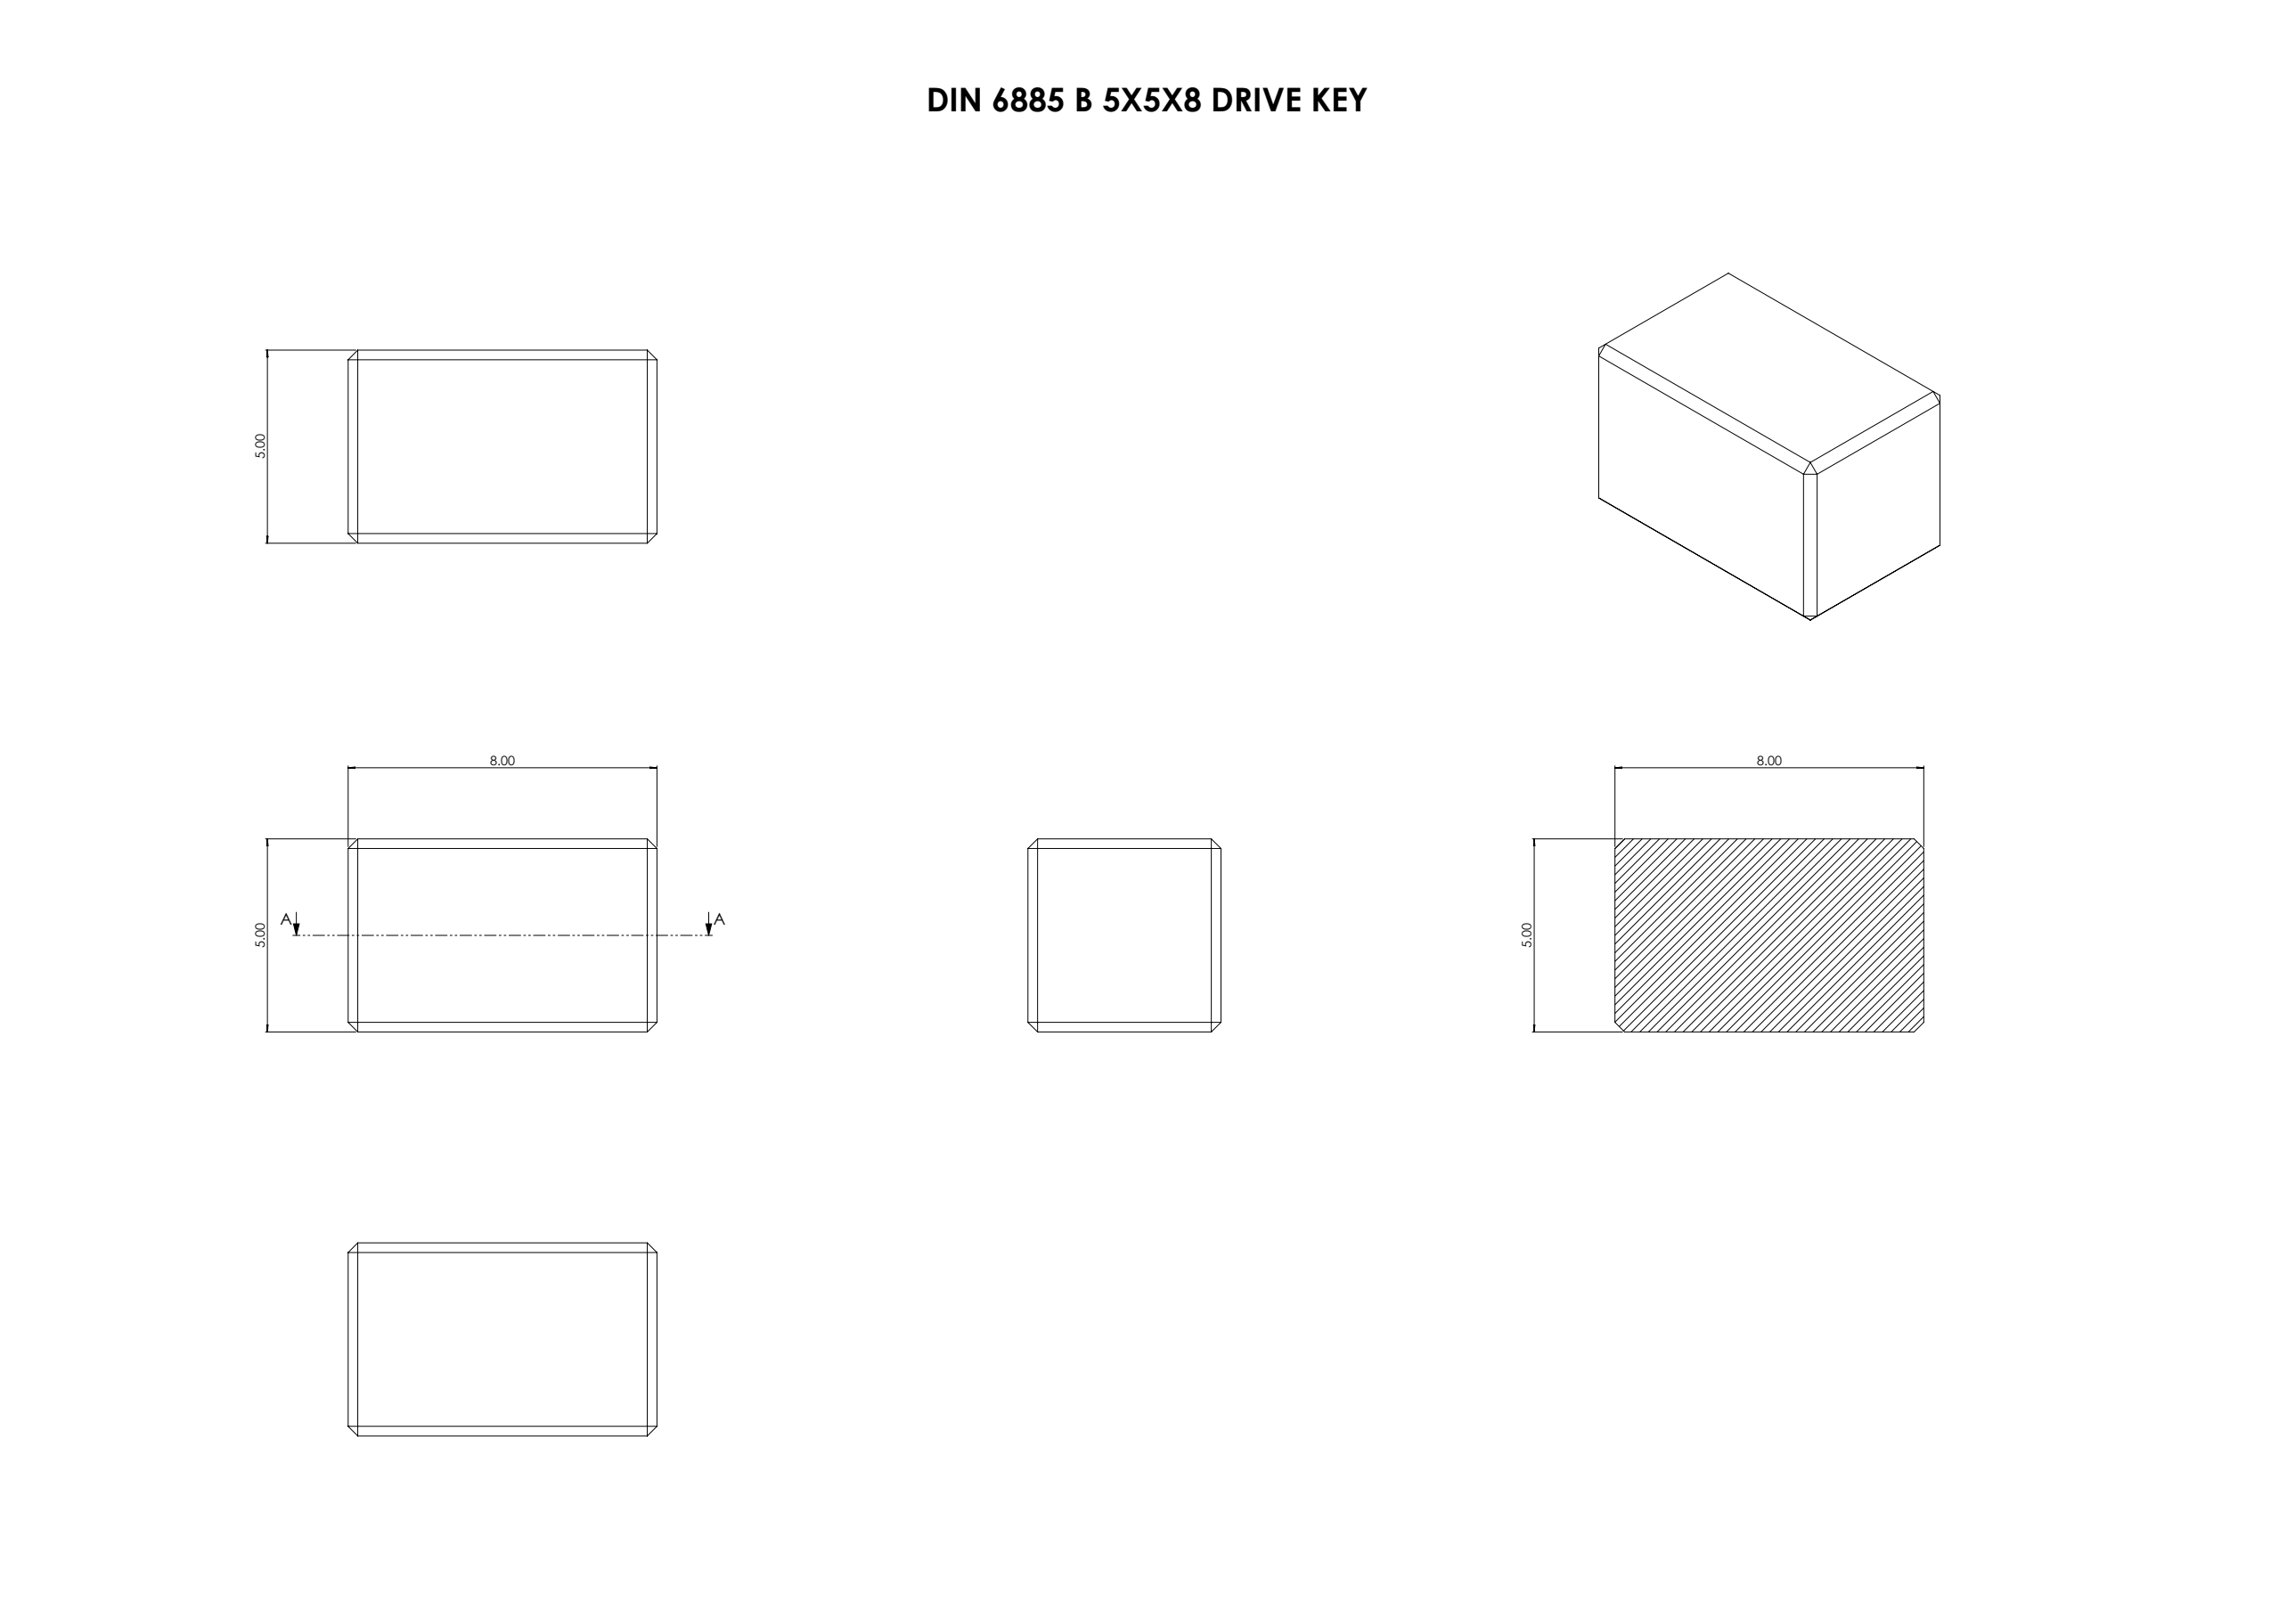
ISO-10303-21;
HEADER;
/* Generated by software containing ST-Developer
 * from STEP Tools, Inc. (www.steptools.com) 
 */

FILE_DESCRIPTION(
/* description */ (''),
/* implementation_level */ '2;1');

FILE_NAME(
/* name */ '10_DIN_6885_B_5x5x8_Drive_Key.step',
/* time_stamp */ '2026-10-24T13:41:11-07:00',
/* author */ (''),
/* organization */ (''),
/* preprocessor_version */ 'ST-DEVELOPER v20.2',
/* originating_system */ 'Autodesk Translation Framework v15.15.0.0',
/* authorisation */ '');

FILE_SCHEMA (('AUTOMOTIVE_DESIGN { 1 0 10303 214 3 1 1 }'));
ENDSEC;

DATA;
#10=MECHANICAL_DESIGN_GEOMETRIC_PRESENTATION_REPRESENTATION('',(#130),#12813);
#110=SHAPE_REPRESENTATION_RELATIONSHIP('SRR','None',#12863,#120);
#120=ADVANCED_BREP_SHAPE_REPRESENTATION('',(#140),#12812);
#130=STYLED_ITEM('',(#12974),#140);
#140=MANIFOLD_SOLID_BREP('Body1',#4393);
#232=PLANE('',#4965);
#233=PLANE('',#4966);
#234=PLANE('',#4967);
#235=PLANE('',#4968);
#236=PLANE('',#4969);
#237=PLANE('',#4970);
#238=PLANE('',#4971);
#239=PLANE('',#4972);
#240=PLANE('',#4973);
#241=PLANE('',#4974);
#242=PLANE('',#4975);
#243=PLANE('',#4976);
#244=PLANE('',#4977);
#245=PLANE('',#4978);
#246=PLANE('',#4979);
#247=PLANE('',#4980);
#248=PLANE('',#4981);
#249=PLANE('',#4982);
#250=PLANE('',#4983);
#251=PLANE('',#4984);
#252=PLANE('',#4985);
#253=PLANE('',#4986);
#254=PLANE('',#4987);
#255=PLANE('',#4988);
#256=PLANE('',#4989);
#257=PLANE('',#4990);
#568=FACE_OUTER_BOUND('',#866,.T.);
#569=FACE_OUTER_BOUND('',#867,.T.);
#570=FACE_OUTER_BOUND('',#868,.T.);
#571=FACE_OUTER_BOUND('',#869,.T.);
#572=FACE_OUTER_BOUND('',#870,.T.);
#573=FACE_OUTER_BOUND('',#871,.T.);
#574=FACE_OUTER_BOUND('',#872,.T.);
#575=FACE_OUTER_BOUND('',#873,.T.);
#576=FACE_OUTER_BOUND('',#874,.T.);
#577=FACE_OUTER_BOUND('',#875,.T.);
#578=FACE_OUTER_BOUND('',#876,.T.);
#579=FACE_OUTER_BOUND('',#877,.T.);
#580=FACE_OUTER_BOUND('',#878,.T.);
#581=FACE_OUTER_BOUND('',#879,.T.);
#582=FACE_OUTER_BOUND('',#880,.T.);
#583=FACE_OUTER_BOUND('',#881,.T.);
#584=FACE_OUTER_BOUND('',#882,.T.);
#585=FACE_OUTER_BOUND('',#883,.T.);
#586=FACE_OUTER_BOUND('',#884,.T.);
#587=FACE_OUTER_BOUND('',#885,.T.);
#588=FACE_OUTER_BOUND('',#886,.T.);
#589=FACE_OUTER_BOUND('',#887,.T.);
#590=FACE_OUTER_BOUND('',#888,.T.);
#591=FACE_OUTER_BOUND('',#889,.T.);
#592=FACE_OUTER_BOUND('',#890,.T.);
#593=FACE_OUTER_BOUND('',#891,.T.);
#866=EDGE_LOOP('',(#3933,#3934,#3935));
#867=EDGE_LOOP('',(#3936,#3937,#3938));
#868=EDGE_LOOP('',(#3939,#3940,#3941));
#869=EDGE_LOOP('',(#3942,#3943,#3944));
#870=EDGE_LOOP('',(#3945,#3946,#3947,#3948));
#871=EDGE_LOOP('',(#3949,#3950,#3951));
#872=EDGE_LOOP('',(#3952,#3953,#3954));
#873=EDGE_LOOP('',(#3955,#3956,#3957,#3958));
#874=EDGE_LOOP('',(#3959,#3960,#3961));
#875=EDGE_LOOP('',(#3962,#3963,#3964,#3965));
#876=EDGE_LOOP('',(#3966,#3967,#3968,#3969));
#877=EDGE_LOOP('',(#3970,#3971,#3972));
#878=EDGE_LOOP('',(#3973,#3974,#3975,#3976));
#879=EDGE_LOOP('',(#3977,#3978,#3979,#3980));
#880=EDGE_LOOP('',(#3981,#3982,#3983,#3984));
#881=EDGE_LOOP('',(#3985,#3986,#3987,#3988));
#882=EDGE_LOOP('',(#3989,#3990,#3991,#3992));
#883=EDGE_LOOP('',(#3993,#3994,#3995,#3996));
#884=EDGE_LOOP('',(#3997,#3998,#3999,#4000));
#885=EDGE_LOOP('',(#4001,#4002,#4003,#4004));
#886=EDGE_LOOP('',(#4005,#4006,#4007,#4008));
#887=EDGE_LOOP('',(#4009,#4010,#4011,#4012));
#888=EDGE_LOOP('',(#4013,#4014,#4015,#4016));
#889=EDGE_LOOP('',(#4017,#4018,#4019,#4020));
#890=EDGE_LOOP('',(#4021,#4022,#4023,#4024));
#891=EDGE_LOOP('',(#4025,#4026,#4027,#4028));
#1305=LINE('',#12682,#1535);
#1306=LINE('',#12684,#1536);
#1307=LINE('',#12685,#1537);
#1308=LINE('',#12689,#1538);
#1309=LINE('',#12691,#1539);
#1310=LINE('',#12692,#1540);
#1311=LINE('',#12696,#1541);
#1312=LINE('',#12698,#1542);
#1313=LINE('',#12699,#1543);
#1314=LINE('',#12703,#1544);
#1315=LINE('',#12705,#1545);
#1316=LINE('',#12706,#1546);
#1317=LINE('',#12708,#1547);
#1318=LINE('',#12709,#1548);
#1319=LINE('',#12713,#1549);
#1320=LINE('',#12715,#1550);
#1321=LINE('',#12716,#1551);
#1322=LINE('',#12720,#1552);
#1323=LINE('',#12722,#1553);
#1324=LINE('',#12723,#1554);
#1325=LINE('',#12725,#1555);
#1326=LINE('',#12726,#1556);
#1327=LINE('',#12730,#1557);
#1328=LINE('',#12732,#1558);
#1329=LINE('',#12733,#1559);
#1330=LINE('',#12735,#1560);
#1331=LINE('',#12736,#1561);
#1332=LINE('',#12738,#1562);
#1333=LINE('',#12739,#1563);
#1334=LINE('',#12743,#1564);
#1335=LINE('',#12745,#1565);
#1336=LINE('',#12746,#1566);
#1337=LINE('',#12748,#1567);
#1338=LINE('',#12749,#1568);
#1339=LINE('',#12751,#1569);
#1340=LINE('',#12752,#1570);
#1341=LINE('',#12754,#1571);
#1342=LINE('',#12755,#1572);
#1343=LINE('',#12757,#1573);
#1344=LINE('',#12758,#1574);
#1345=LINE('',#12760,#1575);
#1346=LINE('',#12761,#1576);
#1347=LINE('',#12763,#1577);
#1348=LINE('',#12764,#1578);
#1349=LINE('',#12766,#1579);
#1350=LINE('',#12767,#1580);
#1351=LINE('',#12769,#1581);
#1352=LINE('',#12770,#1582);
#1535=VECTOR('',#6108,10.);
#1536=VECTOR('',#6109,10.);
#1537=VECTOR('',#6110,10.);
#1538=VECTOR('',#6113,10.);
#1539=VECTOR('',#6114,10.);
#1540=VECTOR('',#6115,10.);
#1541=VECTOR('',#6118,10.);
#1542=VECTOR('',#6119,10.);
#1543=VECTOR('',#6120,10.);
#1544=VECTOR('',#6123,10.);
#1545=VECTOR('',#6124,10.);
#1546=VECTOR('',#6125,10.);
#1547=VECTOR('',#6128,10.);
#1548=VECTOR('',#6129,10.);
#1549=VECTOR('',#6132,10.);
#1550=VECTOR('',#6133,10.);
#1551=VECTOR('',#6134,10.);
#1552=VECTOR('',#6137,10.);
#1553=VECTOR('',#6138,10.);
#1554=VECTOR('',#6139,10.);
#1555=VECTOR('',#6142,10.);
#1556=VECTOR('',#6143,10.);
#1557=VECTOR('',#6146,10.);
#1558=VECTOR('',#6147,10.);
#1559=VECTOR('',#6148,10.);
#1560=VECTOR('',#6151,10.);
#1561=VECTOR('',#6152,10.);
#1562=VECTOR('',#6155,10.);
#1563=VECTOR('',#6156,10.);
#1564=VECTOR('',#6159,10.);
#1565=VECTOR('',#6160,10.);
#1566=VECTOR('',#6161,10.);
#1567=VECTOR('',#6164,10.);
#1568=VECTOR('',#6165,10.);
#1569=VECTOR('',#6168,10.);
#1570=VECTOR('',#6169,10.);
#1571=VECTOR('',#6172,10.);
#1572=VECTOR('',#6173,10.);
#1573=VECTOR('',#6176,10.);
#1574=VECTOR('',#6177,10.);
#1575=VECTOR('',#6180,10.);
#1576=VECTOR('',#6181,10.);
#1577=VECTOR('',#6184,10.);
#1578=VECTOR('',#6185,10.);
#1579=VECTOR('',#6188,10.);
#1580=VECTOR('',#6189,10.);
#1581=VECTOR('',#6192,10.);
#1582=VECTOR('',#6193,10.);
#2112=VERTEX_POINT('',#12680);
#2113=VERTEX_POINT('',#12681);
#2114=VERTEX_POINT('',#12683);
#2115=VERTEX_POINT('',#12687);
#2116=VERTEX_POINT('',#12688);
#2117=VERTEX_POINT('',#12690);
#2118=VERTEX_POINT('',#12694);
#2119=VERTEX_POINT('',#12695);
#2120=VERTEX_POINT('',#12697);
#2121=VERTEX_POINT('',#12701);
#2122=VERTEX_POINT('',#12702);
#2123=VERTEX_POINT('',#12704);
#2124=VERTEX_POINT('',#12711);
#2125=VERTEX_POINT('',#12712);
#2126=VERTEX_POINT('',#12714);
#2127=VERTEX_POINT('',#12718);
#2128=VERTEX_POINT('',#12719);
#2129=VERTEX_POINT('',#12721);
#2130=VERTEX_POINT('',#12728);
#2131=VERTEX_POINT('',#12729);
#2132=VERTEX_POINT('',#12731);
#2133=VERTEX_POINT('',#12741);
#2134=VERTEX_POINT('',#12742);
#2135=VERTEX_POINT('',#12744);
#2719=EDGE_CURVE('',#2112,#2113,#1305,.T.);
#2720=EDGE_CURVE('',#2114,#2112,#1306,.T.);
#2721=EDGE_CURVE('',#2113,#2114,#1307,.T.);
#2722=EDGE_CURVE('',#2115,#2116,#1308,.T.);
#2723=EDGE_CURVE('',#2117,#2115,#1309,.T.);
#2724=EDGE_CURVE('',#2116,#2117,#1310,.T.);
#2725=EDGE_CURVE('',#2118,#2119,#1311,.T.);
#2726=EDGE_CURVE('',#2120,#2118,#1312,.T.);
#2727=EDGE_CURVE('',#2119,#2120,#1313,.T.);
#2728=EDGE_CURVE('',#2121,#2122,#1314,.T.);
#2729=EDGE_CURVE('',#2123,#2121,#1315,.T.);
#2730=EDGE_CURVE('',#2122,#2123,#1316,.T.);
#2731=EDGE_CURVE('',#2112,#2123,#1317,.T.);
#2732=EDGE_CURVE('',#2121,#2114,#1318,.T.);
#2733=EDGE_CURVE('',#2124,#2125,#1319,.T.);
#2734=EDGE_CURVE('',#2126,#2124,#1320,.T.);
#2735=EDGE_CURVE('',#2125,#2126,#1321,.T.);
#2736=EDGE_CURVE('',#2127,#2128,#1322,.T.);
#2737=EDGE_CURVE('',#2129,#2127,#1323,.T.);
#2738=EDGE_CURVE('',#2128,#2129,#1324,.T.);
#2739=EDGE_CURVE('',#2115,#2129,#1325,.T.);
#2740=EDGE_CURVE('',#2127,#2117,#1326,.T.);
#2741=EDGE_CURVE('',#2130,#2131,#1327,.T.);
#2742=EDGE_CURVE('',#2132,#2130,#1328,.T.);
#2743=EDGE_CURVE('',#2131,#2132,#1329,.T.);
#2744=EDGE_CURVE('',#2130,#2120,#1330,.T.);
#2745=EDGE_CURVE('',#2118,#2132,#1331,.T.);
#2746=EDGE_CURVE('',#2122,#2131,#1332,.T.);
#2747=EDGE_CURVE('',#2132,#2121,#1333,.T.);
#2748=EDGE_CURVE('',#2133,#2134,#1334,.T.);
#2749=EDGE_CURVE('',#2135,#2133,#1335,.T.);
#2750=EDGE_CURVE('',#2134,#2135,#1336,.T.);
#2751=EDGE_CURVE('',#2124,#2135,#1337,.T.);
#2752=EDGE_CURVE('',#2133,#2126,#1338,.T.);
#2753=EDGE_CURVE('',#2131,#2134,#1339,.T.);
#2754=EDGE_CURVE('',#2135,#2130,#1340,.T.);
#2755=EDGE_CURVE('',#2134,#2128,#1341,.T.);
#2756=EDGE_CURVE('',#2129,#2133,#1342,.T.);
#2757=EDGE_CURVE('',#2128,#2122,#1343,.T.);
#2758=EDGE_CURVE('',#2123,#2127,#1344,.T.);
#2759=EDGE_CURVE('',#2116,#2125,#1345,.T.);
#2760=EDGE_CURVE('',#2126,#2115,#1346,.T.);
#2761=EDGE_CURVE('',#2125,#2119,#1347,.T.);
#2762=EDGE_CURVE('',#2120,#2124,#1348,.T.);
#2763=EDGE_CURVE('',#2119,#2113,#1349,.T.);
#2764=EDGE_CURVE('',#2114,#2118,#1350,.T.);
#2765=EDGE_CURVE('',#2113,#2116,#1351,.T.);
#2766=EDGE_CURVE('',#2117,#2112,#1352,.T.);
#3933=ORIENTED_EDGE('',*,*,#2719,.F.);
#3934=ORIENTED_EDGE('',*,*,#2720,.F.);
#3935=ORIENTED_EDGE('',*,*,#2721,.F.);
#3936=ORIENTED_EDGE('',*,*,#2722,.F.);
#3937=ORIENTED_EDGE('',*,*,#2723,.F.);
#3938=ORIENTED_EDGE('',*,*,#2724,.F.);
#3939=ORIENTED_EDGE('',*,*,#2725,.F.);
#3940=ORIENTED_EDGE('',*,*,#2726,.F.);
#3941=ORIENTED_EDGE('',*,*,#2727,.F.);
#3942=ORIENTED_EDGE('',*,*,#2728,.F.);
#3943=ORIENTED_EDGE('',*,*,#2729,.F.);
#3944=ORIENTED_EDGE('',*,*,#2730,.F.);
#3945=ORIENTED_EDGE('',*,*,#2720,.T.);
#3946=ORIENTED_EDGE('',*,*,#2731,.T.);
#3947=ORIENTED_EDGE('',*,*,#2729,.T.);
#3948=ORIENTED_EDGE('',*,*,#2732,.T.);
#3949=ORIENTED_EDGE('',*,*,#2733,.F.);
#3950=ORIENTED_EDGE('',*,*,#2734,.F.);
#3951=ORIENTED_EDGE('',*,*,#2735,.F.);
#3952=ORIENTED_EDGE('',*,*,#2736,.F.);
#3953=ORIENTED_EDGE('',*,*,#2737,.F.);
#3954=ORIENTED_EDGE('',*,*,#2738,.F.);
#3955=ORIENTED_EDGE('',*,*,#2723,.T.);
#3956=ORIENTED_EDGE('',*,*,#2739,.T.);
#3957=ORIENTED_EDGE('',*,*,#2737,.T.);
#3958=ORIENTED_EDGE('',*,*,#2740,.T.);
#3959=ORIENTED_EDGE('',*,*,#2741,.F.);
#3960=ORIENTED_EDGE('',*,*,#2742,.F.);
#3961=ORIENTED_EDGE('',*,*,#2743,.F.);
#3962=ORIENTED_EDGE('',*,*,#2742,.T.);
#3963=ORIENTED_EDGE('',*,*,#2744,.T.);
#3964=ORIENTED_EDGE('',*,*,#2726,.T.);
#3965=ORIENTED_EDGE('',*,*,#2745,.T.);
#3966=ORIENTED_EDGE('',*,*,#2728,.T.);
#3967=ORIENTED_EDGE('',*,*,#2746,.T.);
#3968=ORIENTED_EDGE('',*,*,#2743,.T.);
#3969=ORIENTED_EDGE('',*,*,#2747,.T.);
#3970=ORIENTED_EDGE('',*,*,#2748,.F.);
#3971=ORIENTED_EDGE('',*,*,#2749,.F.);
#3972=ORIENTED_EDGE('',*,*,#2750,.F.);
#3973=ORIENTED_EDGE('',*,*,#2734,.T.);
#3974=ORIENTED_EDGE('',*,*,#2751,.T.);
#3975=ORIENTED_EDGE('',*,*,#2749,.T.);
#3976=ORIENTED_EDGE('',*,*,#2752,.T.);
#3977=ORIENTED_EDGE('',*,*,#2741,.T.);
#3978=ORIENTED_EDGE('',*,*,#2753,.T.);
#3979=ORIENTED_EDGE('',*,*,#2750,.T.);
#3980=ORIENTED_EDGE('',*,*,#2754,.T.);
#3981=ORIENTED_EDGE('',*,*,#2748,.T.);
#3982=ORIENTED_EDGE('',*,*,#2755,.T.);
#3983=ORIENTED_EDGE('',*,*,#2738,.T.);
#3984=ORIENTED_EDGE('',*,*,#2756,.T.);
#3985=ORIENTED_EDGE('',*,*,#2736,.T.);
#3986=ORIENTED_EDGE('',*,*,#2757,.T.);
#3987=ORIENTED_EDGE('',*,*,#2730,.T.);
#3988=ORIENTED_EDGE('',*,*,#2758,.T.);
#3989=ORIENTED_EDGE('',*,*,#2722,.T.);
#3990=ORIENTED_EDGE('',*,*,#2759,.T.);
#3991=ORIENTED_EDGE('',*,*,#2735,.T.);
#3992=ORIENTED_EDGE('',*,*,#2760,.T.);
#3993=ORIENTED_EDGE('',*,*,#2733,.T.);
#3994=ORIENTED_EDGE('',*,*,#2761,.T.);
#3995=ORIENTED_EDGE('',*,*,#2727,.T.);
#3996=ORIENTED_EDGE('',*,*,#2762,.T.);
#3997=ORIENTED_EDGE('',*,*,#2725,.T.);
#3998=ORIENTED_EDGE('',*,*,#2763,.T.);
#3999=ORIENTED_EDGE('',*,*,#2721,.T.);
#4000=ORIENTED_EDGE('',*,*,#2764,.T.);
#4001=ORIENTED_EDGE('',*,*,#2719,.T.);
#4002=ORIENTED_EDGE('',*,*,#2765,.T.);
#4003=ORIENTED_EDGE('',*,*,#2724,.T.);
#4004=ORIENTED_EDGE('',*,*,#2766,.T.);
#4005=ORIENTED_EDGE('',*,*,#2740,.F.);
#4006=ORIENTED_EDGE('',*,*,#2758,.F.);
#4007=ORIENTED_EDGE('',*,*,#2731,.F.);
#4008=ORIENTED_EDGE('',*,*,#2766,.F.);
#4009=ORIENTED_EDGE('',*,*,#2745,.F.);
#4010=ORIENTED_EDGE('',*,*,#2764,.F.);
#4011=ORIENTED_EDGE('',*,*,#2732,.F.);
#4012=ORIENTED_EDGE('',*,*,#2747,.F.);
#4013=ORIENTED_EDGE('',*,*,#2746,.F.);
#4014=ORIENTED_EDGE('',*,*,#2757,.F.);
#4015=ORIENTED_EDGE('',*,*,#2755,.F.);
#4016=ORIENTED_EDGE('',*,*,#2753,.F.);
#4017=ORIENTED_EDGE('',*,*,#2752,.F.);
#4018=ORIENTED_EDGE('',*,*,#2756,.F.);
#4019=ORIENTED_EDGE('',*,*,#2739,.F.);
#4020=ORIENTED_EDGE('',*,*,#2760,.F.);
#4021=ORIENTED_EDGE('',*,*,#2751,.F.);
#4022=ORIENTED_EDGE('',*,*,#2762,.F.);
#4023=ORIENTED_EDGE('',*,*,#2744,.F.);
#4024=ORIENTED_EDGE('',*,*,#2754,.F.);
#4025=ORIENTED_EDGE('',*,*,#2759,.F.);
#4026=ORIENTED_EDGE('',*,*,#2765,.F.);
#4027=ORIENTED_EDGE('',*,*,#2763,.F.);
#4028=ORIENTED_EDGE('',*,*,#2761,.F.);
#4358=ADVANCED_FACE('',(#568),#232,.T.);
#4359=ADVANCED_FACE('',(#569),#233,.T.);
#4360=ADVANCED_FACE('',(#570),#234,.T.);
#4361=ADVANCED_FACE('',(#571),#235,.T.);
#4362=ADVANCED_FACE('',(#572),#236,.T.);
#4363=ADVANCED_FACE('',(#573),#237,.T.);
#4364=ADVANCED_FACE('',(#574),#238,.T.);
#4365=ADVANCED_FACE('',(#575),#239,.T.);
#4366=ADVANCED_FACE('',(#576),#240,.T.);
#4367=ADVANCED_FACE('',(#577),#241,.T.);
#4368=ADVANCED_FACE('',(#578),#242,.T.);
#4369=ADVANCED_FACE('',(#579),#243,.T.);
#4370=ADVANCED_FACE('',(#580),#244,.T.);
#4371=ADVANCED_FACE('',(#581),#245,.T.);
#4372=ADVANCED_FACE('',(#582),#246,.T.);
#4373=ADVANCED_FACE('',(#583),#247,.T.);
#4374=ADVANCED_FACE('',(#584),#248,.T.);
#4375=ADVANCED_FACE('',(#585),#249,.T.);
#4376=ADVANCED_FACE('',(#586),#250,.T.);
#4377=ADVANCED_FACE('',(#587),#251,.T.);
#4378=ADVANCED_FACE('',(#588),#252,.T.);
#4379=ADVANCED_FACE('',(#589),#253,.T.);
#4380=ADVANCED_FACE('',(#590),#254,.T.);
#4381=ADVANCED_FACE('',(#591),#255,.T.);
#4382=ADVANCED_FACE('',(#592),#256,.T.);
#4383=ADVANCED_FACE('',(#593),#257,.T.);
#4393=CLOSED_SHELL('',(#4358,#4359,#4360,#4361,#4362,#4363,#4364,#4365,
#4366,#4367,#4368,#4369,#4370,#4371,#4372,#4373,#4374,#4375,#4376,#4377,
#4378,#4379,#4380,#4381,#4382,#4383));
#4964=AXIS2_PLACEMENT_3D('',#12678,#6104,#6105);
#4965=AXIS2_PLACEMENT_3D('',#12679,#6106,#6107);
#4966=AXIS2_PLACEMENT_3D('',#12686,#6111,#6112);
#4967=AXIS2_PLACEMENT_3D('',#12693,#6116,#6117);
#4968=AXIS2_PLACEMENT_3D('',#12700,#6121,#6122);
#4969=AXIS2_PLACEMENT_3D('',#12707,#6126,#6127);
#4970=AXIS2_PLACEMENT_3D('',#12710,#6130,#6131);
#4971=AXIS2_PLACEMENT_3D('',#12717,#6135,#6136);
#4972=AXIS2_PLACEMENT_3D('',#12724,#6140,#6141);
#4973=AXIS2_PLACEMENT_3D('',#12727,#6144,#6145);
#4974=AXIS2_PLACEMENT_3D('',#12734,#6149,#6150);
#4975=AXIS2_PLACEMENT_3D('',#12737,#6153,#6154);
#4976=AXIS2_PLACEMENT_3D('',#12740,#6157,#6158);
#4977=AXIS2_PLACEMENT_3D('',#12747,#6162,#6163);
#4978=AXIS2_PLACEMENT_3D('',#12750,#6166,#6167);
#4979=AXIS2_PLACEMENT_3D('',#12753,#6170,#6171);
#4980=AXIS2_PLACEMENT_3D('',#12756,#6174,#6175);
#4981=AXIS2_PLACEMENT_3D('',#12759,#6178,#6179);
#4982=AXIS2_PLACEMENT_3D('',#12762,#6182,#6183);
#4983=AXIS2_PLACEMENT_3D('',#12765,#6186,#6187);
#4984=AXIS2_PLACEMENT_3D('',#12768,#6190,#6191);
#4985=AXIS2_PLACEMENT_3D('',#12771,#6194,#6195);
#4986=AXIS2_PLACEMENT_3D('',#12772,#6196,#6197);
#4987=AXIS2_PLACEMENT_3D('',#12773,#6198,#6199);
#4988=AXIS2_PLACEMENT_3D('',#12774,#6200,#6201);
#4989=AXIS2_PLACEMENT_3D('',#12775,#6202,#6203);
#4990=AXIS2_PLACEMENT_3D('',#12776,#6204,#6205);
#6104=DIRECTION('axis',(0.,0.,1.));
#6105=DIRECTION('refdir',(1.,0.,0.));
#6106=DIRECTION('center_axis',(0.577350269189626,0.577350269189624,0.577350269189627));
#6107=DIRECTION('ref_axis',(0.707106781186548,0.,-0.707106781186547));
#6108=DIRECTION('',(-0.707106781186548,0.,0.707106781186547));
#6109=DIRECTION('',(0.707106781186546,-0.707106781186549,0.));
#6110=DIRECTION('',(3.14018491736755E-15,0.707106781186548,-0.707106781186547));
#6111=DIRECTION('center_axis',(0.577350269189625,-0.577350269189626,0.577350269189626));
#6112=DIRECTION('ref_axis',(0.707106781186548,0.,-0.707106781186547));
#6113=DIRECTION('',(0.,0.707106781186547,0.707106781186548));
#6114=DIRECTION('',(-0.707106781186548,-0.707106781186547,0.));
#6115=DIRECTION('',(0.707106781186548,0.,-0.707106781186547));
#6116=DIRECTION('center_axis',(-0.577350269189626,0.577350269189626,0.577350269189626));
#6117=DIRECTION('ref_axis',(0.707106781186547,0.,0.707106781186547));
#6118=DIRECTION('',(0.,-0.707106781186548,0.707106781186547));
#6119=DIRECTION('',(0.707106781186547,0.707106781186547,0.));
#6120=DIRECTION('',(-0.707106781186547,0.,-0.707106781186547));
#6121=DIRECTION('center_axis',(0.577350269189626,0.577350269189624,-0.577350269189627));
#6122=DIRECTION('ref_axis',(-0.707106781186548,0.,-0.707106781186547));
#6123=DIRECTION('',(-3.14018491736755E-15,-0.707106781186548,-0.707106781186547));
#6124=DIRECTION('',(-0.707106781186546,0.707106781186549,0.));
#6125=DIRECTION('',(0.707106781186548,0.,0.707106781186547));
#6126=DIRECTION('center_axis',(0.707106781186549,0.707106781186546,0.));
#6127=DIRECTION('ref_axis',(0.,0.,-1.));
#6128=DIRECTION('',(0.,0.,-1.));
#6129=DIRECTION('',(0.,0.,1.));
#6130=DIRECTION('center_axis',(-0.577350269189627,-0.577350269189625,0.577350269189625));
#6131=DIRECTION('ref_axis',(0.707106781186546,0.,0.707106781186549));
#6132=DIRECTION('',(0.707106781186547,-3.14018491736755E-15,0.707106781186547));
#6133=DIRECTION('',(-0.707106781186546,0.707106781186549,0.));
#6134=DIRECTION('',(0.,-0.707106781186547,-0.707106781186548));
#6135=DIRECTION('center_axis',(0.577350269189625,-0.577350269189627,-0.577350269189626));
#6136=DIRECTION('ref_axis',(-0.707106781186548,0.,-0.707106781186547));
#6137=DIRECTION('',(-0.707106781186548,0.,-0.707106781186547));
#6138=DIRECTION('',(0.707106781186548,0.707106781186547,0.));
#6139=DIRECTION('',(0.,-0.707106781186547,0.707106781186548));
#6140=DIRECTION('center_axis',(0.707106781186547,-0.707106781186548,0.));
#6141=DIRECTION('ref_axis',(0.,0.,-1.));
#6142=DIRECTION('',(0.,0.,-1.));
#6143=DIRECTION('',(0.,0.,1.));
#6144=DIRECTION('center_axis',(-0.577350269189626,0.577350269189626,-0.577350269189626));
#6145=DIRECTION('ref_axis',(-0.707106781186548,0.,0.707106781186547));
#6146=DIRECTION('',(0.707106781186547,0.,-0.707106781186547));
#6147=DIRECTION('',(-0.707106781186547,-0.707106781186547,0.));
#6148=DIRECTION('',(0.,0.707106781186548,0.707106781186547));
#6149=DIRECTION('center_axis',(-0.707106781186548,0.707106781186548,0.));
#6150=DIRECTION('ref_axis',(0.,0.,1.));
#6151=DIRECTION('',(0.,0.,1.));
#6152=DIRECTION('',(0.,0.,-1.));
#6153=DIRECTION('center_axis',(0.,0.707106781186547,-0.707106781186548));
#6154=DIRECTION('ref_axis',(-1.,0.,0.));
#6155=DIRECTION('',(-1.,0.,0.));
#6156=DIRECTION('',(1.,0.,0.));
#6157=DIRECTION('center_axis',(-0.577350269189627,-0.577350269189625,-0.577350269189625));
#6158=DIRECTION('ref_axis',(-0.707106781186546,0.,0.707106781186549));
#6159=DIRECTION('',(0.,0.707106781186547,-0.707106781186548));
#6160=DIRECTION('',(0.707106781186546,-0.707106781186549,0.));
#6161=DIRECTION('',(-0.707106781186547,3.14018491736755E-15,0.707106781186547));
#6162=DIRECTION('center_axis',(-0.707106781186549,-0.707106781186546,0.));
#6163=DIRECTION('ref_axis',(0.,0.,1.));
#6164=DIRECTION('',(0.,0.,-1.));
#6165=DIRECTION('',(0.,0.,1.));
#6166=DIRECTION('center_axis',(-0.707106781186548,0.,-0.707106781186548));
#6167=DIRECTION('ref_axis',(-0.707106781186548,0.,0.707106781186548));
#6168=DIRECTION('',(0.,-1.,0.));
#6169=DIRECTION('',(0.,1.,0.));
#6170=DIRECTION('center_axis',(0.,-0.707106781186548,-0.707106781186547));
#6171=DIRECTION('ref_axis',(-1.,0.,0.));
#6172=DIRECTION('',(1.,0.,0.));
#6173=DIRECTION('',(-1.,0.,0.));
#6174=DIRECTION('center_axis',(0.707106781186547,0.,-0.707106781186548));
#6175=DIRECTION('ref_axis',(-0.707106781186548,0.,-0.707106781186547));
#6176=DIRECTION('',(0.,1.,0.));
#6177=DIRECTION('',(0.,-1.,0.));
#6178=DIRECTION('center_axis',(0.,-0.707106781186548,0.707106781186547));
#6179=DIRECTION('ref_axis',(1.,0.,0.));
#6180=DIRECTION('',(-1.,0.,0.));
#6181=DIRECTION('',(1.,0.,0.));
#6182=DIRECTION('center_axis',(-0.707106781186548,0.,0.707106781186548));
#6183=DIRECTION('ref_axis',(0.707106781186548,0.,0.707106781186548));
#6184=DIRECTION('',(0.,1.,0.));
#6185=DIRECTION('',(0.,-1.,0.));
#6186=DIRECTION('center_axis',(0.,0.707106781186547,0.707106781186548));
#6187=DIRECTION('ref_axis',(1.,0.,0.));
#6188=DIRECTION('',(1.,0.,0.));
#6189=DIRECTION('',(-1.,0.,0.));
#6190=DIRECTION('center_axis',(0.707106781186547,0.,0.707106781186548));
#6191=DIRECTION('ref_axis',(0.707106781186548,0.,-0.707106781186547));
#6192=DIRECTION('',(0.,-1.,0.));
#6193=DIRECTION('',(0.,1.,0.));
#6194=DIRECTION('center_axis',(1.,0.,0.));
#6195=DIRECTION('ref_axis',(0.,1.,0.));
#6196=DIRECTION('center_axis',(0.,1.,0.));
#6197=DIRECTION('ref_axis',(-1.,0.,0.));
#6198=DIRECTION('center_axis',(0.,0.,-1.));
#6199=DIRECTION('ref_axis',(-1.,0.,0.));
#6200=DIRECTION('center_axis',(0.,-1.,0.));
#6201=DIRECTION('ref_axis',(1.,0.,0.));
#6202=DIRECTION('center_axis',(-1.,0.,0.));
#6203=DIRECTION('ref_axis',(0.,-1.,0.));
#6204=DIRECTION('center_axis',(0.,0.,1.));
#6205=DIRECTION('ref_axis',(1.,0.,0.));
#12678=CARTESIAN_POINT('',(0.,0.,0.));
#12679=CARTESIAN_POINT('Origin',(7.75,9.94,2.25));
#12680=CARTESIAN_POINT('',(8.,9.69,2.25));
#12681=CARTESIAN_POINT('',(7.75,9.69,2.5));
#12682=CARTESIAN_POINT('',(8.,9.69,2.25));
#12683=CARTESIAN_POINT('',(7.75,9.94,2.25));
#12684=CARTESIAN_POINT('',(7.75,9.94,2.25));
#12685=CARTESIAN_POINT('',(7.75,9.69,2.5));
#12686=CARTESIAN_POINT('Origin',(8.,5.19,2.25));
#12687=CARTESIAN_POINT('',(7.75,4.94,2.25));
#12688=CARTESIAN_POINT('',(7.75,5.19,2.5));
#12689=CARTESIAN_POINT('',(7.75,4.94,2.25));
#12690=CARTESIAN_POINT('',(8.,5.19,2.25));
#12691=CARTESIAN_POINT('',(8.,5.19,2.25));
#12692=CARTESIAN_POINT('',(7.75,5.19,2.5));
#12693=CARTESIAN_POINT('Origin',(0.,9.69,2.25));
#12694=CARTESIAN_POINT('',(0.25,9.94,2.25));
#12695=CARTESIAN_POINT('',(0.25,9.69,2.5));
#12696=CARTESIAN_POINT('',(0.25,9.94,2.25));
#12697=CARTESIAN_POINT('',(0.,9.69,2.25));
#12698=CARTESIAN_POINT('',(0.,9.69,2.25));
#12699=CARTESIAN_POINT('',(0.25,9.69,2.5));
#12700=CARTESIAN_POINT('Origin',(8.,9.69,-2.25));
#12701=CARTESIAN_POINT('',(7.75,9.94,-2.25));
#12702=CARTESIAN_POINT('',(7.75,9.69,-2.5));
#12703=CARTESIAN_POINT('',(7.75,9.94,-2.25));
#12704=CARTESIAN_POINT('',(8.,9.69,-2.25));
#12705=CARTESIAN_POINT('',(8.,9.69,-2.25));
#12706=CARTESIAN_POINT('',(7.75,9.69,-2.5));
#12707=CARTESIAN_POINT('Origin',(7.875,9.815,0.));
#12708=CARTESIAN_POINT('',(8.,9.69,0.));
#12709=CARTESIAN_POINT('',(7.75,9.94,0.));
#12710=CARTESIAN_POINT('Origin',(0.25,4.94,2.25));
#12711=CARTESIAN_POINT('',(0.,5.19,2.25));
#12712=CARTESIAN_POINT('',(0.25,5.19,2.5));
#12713=CARTESIAN_POINT('',(0.,5.19,2.25));
#12714=CARTESIAN_POINT('',(0.25,4.94,2.25));
#12715=CARTESIAN_POINT('',(0.25,4.94,2.25));
#12716=CARTESIAN_POINT('',(0.25,5.19,2.5));
#12717=CARTESIAN_POINT('Origin',(7.75,4.94,-2.25));
#12718=CARTESIAN_POINT('',(8.,5.19,-2.25));
#12719=CARTESIAN_POINT('',(7.75,5.19,-2.5));
#12720=CARTESIAN_POINT('',(8.,5.19,-2.25));
#12721=CARTESIAN_POINT('',(7.75,4.94,-2.25));
#12722=CARTESIAN_POINT('',(7.75,4.94,-2.25));
#12723=CARTESIAN_POINT('',(7.75,5.19,-2.5));
#12724=CARTESIAN_POINT('Origin',(7.875,5.065,0.));
#12725=CARTESIAN_POINT('',(7.75,4.94,0.));
#12726=CARTESIAN_POINT('',(8.,5.19,0.));
#12727=CARTESIAN_POINT('Origin',(0.25,9.94,-2.25));
#12728=CARTESIAN_POINT('',(0.,9.69,-2.25));
#12729=CARTESIAN_POINT('',(0.25,9.69,-2.5));
#12730=CARTESIAN_POINT('',(0.,9.69,-2.25));
#12731=CARTESIAN_POINT('',(0.25,9.94,-2.25));
#12732=CARTESIAN_POINT('',(0.25,9.94,-2.25));
#12733=CARTESIAN_POINT('',(0.25,9.69,-2.5));
#12734=CARTESIAN_POINT('Origin',(0.125,9.815,0.));
#12735=CARTESIAN_POINT('',(0.,9.69,0.));
#12736=CARTESIAN_POINT('',(0.25,9.94,0.));
#12737=CARTESIAN_POINT('Origin',(6.,9.815,-2.375));
#12738=CARTESIAN_POINT('',(6.,9.69,-2.5));
#12739=CARTESIAN_POINT('',(6.,9.94,-2.25));
#12740=CARTESIAN_POINT('Origin',(0.,5.19,-2.25));
#12741=CARTESIAN_POINT('',(0.25,4.94,-2.25));
#12742=CARTESIAN_POINT('',(0.25,5.19,-2.5));
#12743=CARTESIAN_POINT('',(0.25,4.94,-2.25));
#12744=CARTESIAN_POINT('',(0.,5.19,-2.25));
#12745=CARTESIAN_POINT('',(0.,5.19,-2.25));
#12746=CARTESIAN_POINT('',(0.25,5.19,-2.5));
#12747=CARTESIAN_POINT('Origin',(0.125,5.065,0.));
#12748=CARTESIAN_POINT('',(0.,5.19,0.));
#12749=CARTESIAN_POINT('',(0.25,4.94,0.));
#12750=CARTESIAN_POINT('Origin',(0.125,8.69,-2.375));
#12751=CARTESIAN_POINT('',(0.25,8.69,-2.5));
#12752=CARTESIAN_POINT('',(0.,8.69,-2.25));
#12753=CARTESIAN_POINT('Origin',(2.,5.065,-2.375));
#12754=CARTESIAN_POINT('',(2.,5.19,-2.5));
#12755=CARTESIAN_POINT('',(2.,4.94,-2.25));
#12756=CARTESIAN_POINT('Origin',(7.875,6.19,-2.375));
#12757=CARTESIAN_POINT('',(7.75,6.19,-2.5));
#12758=CARTESIAN_POINT('',(8.,6.19,-2.25));
#12759=CARTESIAN_POINT('Origin',(2.,5.065,2.375));
#12760=CARTESIAN_POINT('',(2.,5.19,2.5));
#12761=CARTESIAN_POINT('',(2.,4.94,2.25));
#12762=CARTESIAN_POINT('Origin',(0.125,8.69,2.375));
#12763=CARTESIAN_POINT('',(0.25,8.69,2.5));
#12764=CARTESIAN_POINT('',(0.,8.69,2.25));
#12765=CARTESIAN_POINT('Origin',(6.,9.815,2.375));
#12766=CARTESIAN_POINT('',(6.,9.69,2.5));
#12767=CARTESIAN_POINT('',(6.,9.94,2.25));
#12768=CARTESIAN_POINT('Origin',(7.875,6.19,2.375));
#12769=CARTESIAN_POINT('',(7.75,6.19,2.5));
#12770=CARTESIAN_POINT('',(8.,6.19,2.25));
#12771=CARTESIAN_POINT('Origin',(8.,4.94,0.));
#12772=CARTESIAN_POINT('Origin',(8.,9.94,0.));
#12773=CARTESIAN_POINT('Origin',(4.,7.44,-2.5));
#12774=CARTESIAN_POINT('Origin',(0.,4.94,0.));
#12775=CARTESIAN_POINT('Origin',(0.,9.94,0.));
#12776=CARTESIAN_POINT('Origin',(4.,7.44,2.5));
#12800=UNCERTAINTY_MEASURE_WITH_UNIT(LENGTH_MEASURE(0.01),#12814,
'DISTANCE_ACCURACY_VALUE',
'Maximum model space distance between geometric entities at asserted c
onnectivities');
#12801=UNCERTAINTY_MEASURE_WITH_UNIT(LENGTH_MEASURE(0.01),#12814,
'DISTANCE_ACCURACY_VALUE',
'Maximum model space distance between geometric entities at asserted c
onnectivities');
#12812=(
GEOMETRIC_REPRESENTATION_CONTEXT(3)
GLOBAL_UNCERTAINTY_ASSIGNED_CONTEXT((#12800))
GLOBAL_UNIT_ASSIGNED_CONTEXT((#12814,#12816,#12817))
REPRESENTATION_CONTEXT('','3D')
);
#12813=(
GEOMETRIC_REPRESENTATION_CONTEXT(3)
GLOBAL_UNCERTAINTY_ASSIGNED_CONTEXT((#12801))
GLOBAL_UNIT_ASSIGNED_CONTEXT((#12814,#12816,#12817))
REPRESENTATION_CONTEXT('','3D')
);
#12814=(
LENGTH_UNIT()
NAMED_UNIT(*)
SI_UNIT(.MILLI.,.METRE.)
);
#12816=(
NAMED_UNIT(*)
PLANE_ANGLE_UNIT()
SI_UNIT($,.RADIAN.)
);
#12817=(
NAMED_UNIT(*)
SI_UNIT($,.STERADIAN.)
SOLID_ANGLE_UNIT()
);
#12828=SHAPE_DEFINITION_REPRESENTATION(#12839,#12863);
#12839=PRODUCT_DEFINITION_SHAPE('',$,#12875);
#12863=SHAPE_REPRESENTATION('',(#4964),#12812);
#12864=PRODUCT_DEFINITION_CONTEXT('part definition',#12899,'design');
#12875=PRODUCT_DEFINITION('2026-10-11-12-17-36-792',
'10_DIN_6885_B_5x5x8_Drive_Key',#12886,#12864);
#12886=PRODUCT_DEFINITION_FORMATION('',$,#12911);
#12899=APPLICATION_CONTEXT(
'Core Data for Automotive Mechanical Design Process');
#12900=PRODUCT_CONTEXT('part definition',#12899,'mechanical');
#12911=PRODUCT('2026-10-11-12-17-36-792',
'10_DIN_6885_B_5x5x8_Drive_Key',$,(#12900));
#12968=COLOUR_RGB('Grey',0.48,0.52,0.57);
#12969=FILL_AREA_STYLE_COLOUR('',#12968);
#12970=FILL_AREA_STYLE('',(#12969));
#12971=SURFACE_STYLE_FILL_AREA(#12970);
#12972=SURFACE_SIDE_STYLE('',(#12971));
#12973=SURFACE_STYLE_USAGE(.BOTH.,#12972);
#12974=PRESENTATION_STYLE_ASSIGNMENT((#12973));
ENDSEC;
END-ISO-10303-21;
